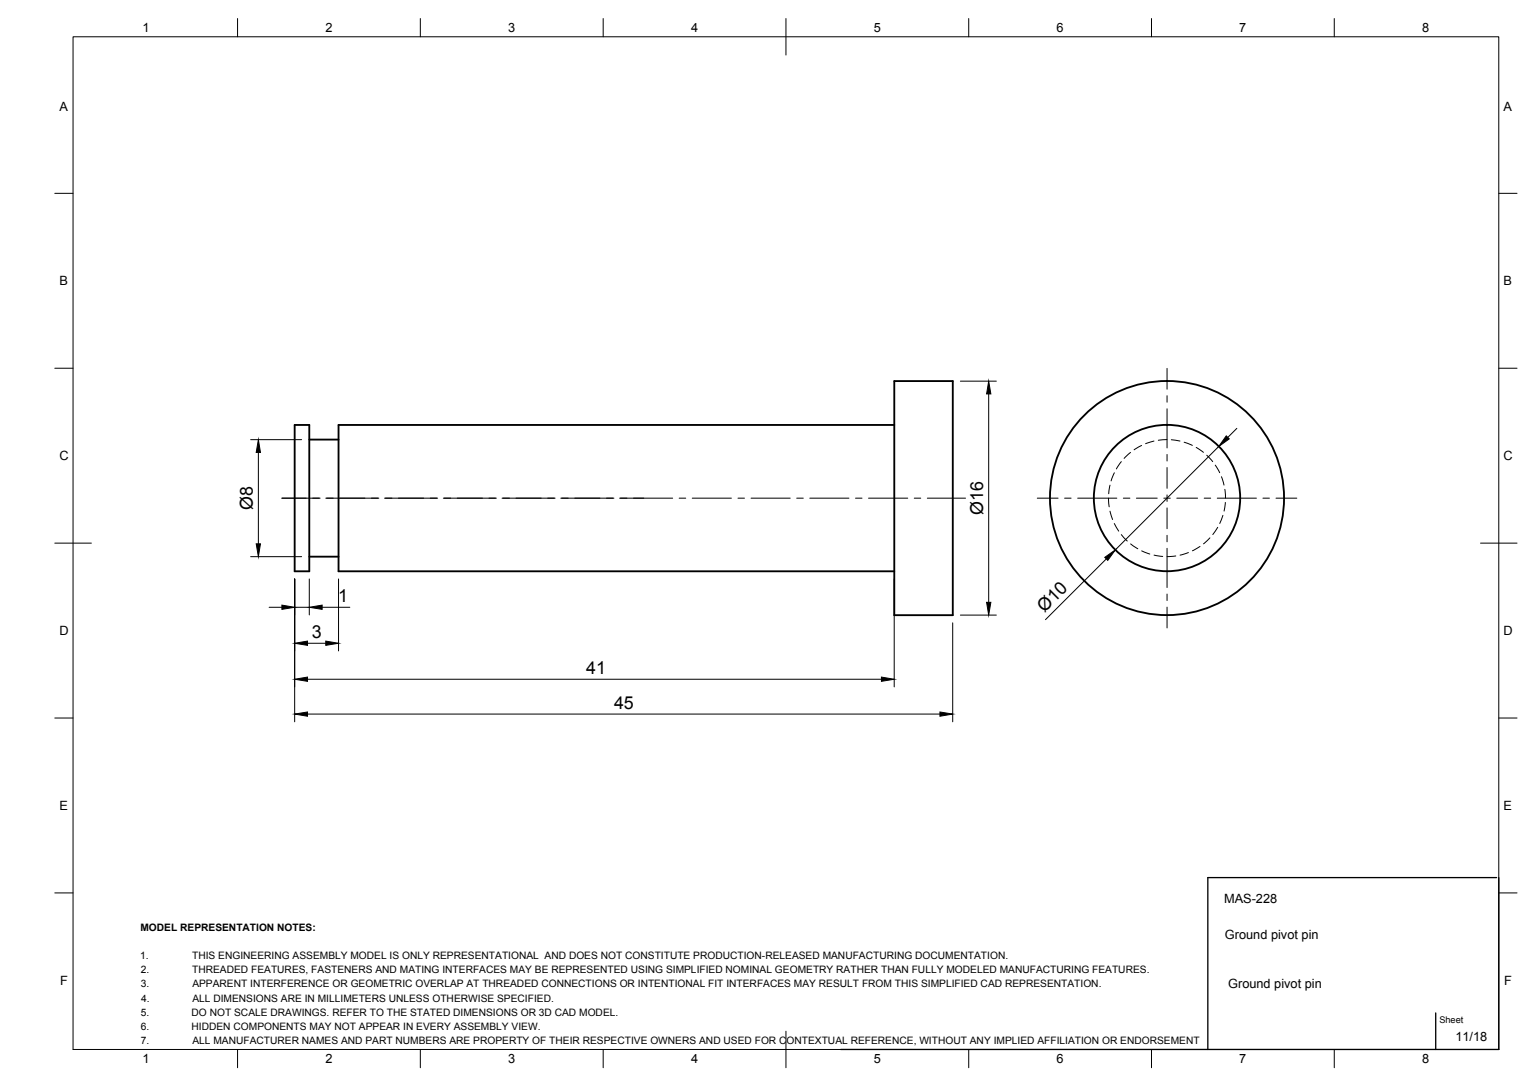
ISO-10303-21;
HEADER;
/* Generated by software containing ST-Developer
 * from STEP Tools, Inc. (www.steptools.com) 
 */

FILE_DESCRIPTION(
/* description */ ('Independent Peaucellier-Lipkin straight-line linkage. Radius arms 100
 mm, inversion-cell links 60 mm, crank radius and fixed-pivot spacing 
32 mm. Inversion constant 6400 mm squared, nominal output straight lin
e X=100 mm. Overhead bearing bridge clears the layered moving links. N
o accuracy or load rating assigned.'),
/* implementation_level */ '2;1');

FILE_NAME(
/* name */ 'Ground pivot pin.step',
/* time_stamp */ '2026-11-09T18:06:16-08:00',
/* author */ (''),
/* organization */ (''),
/* preprocessor_version */ 'ST-DEVELOPER v20.2',
/* originating_system */ 'Autodesk Translation Framework v15.17.0.0',
/* authorisation */ '');

FILE_SCHEMA (('AUTOMOTIVE_DESIGN { 1 0 10303 214 3 1 1 }'));
ENDSEC;

DATA;
#10=MECHANICAL_DESIGN_GEOMETRIC_PRESENTATION_REPRESENTATION('',(#289),#3581);
#255=SHAPE_REPRESENTATION_RELATIONSHIP('SRR','None',#3689,#272);
#272=ADVANCED_BREP_SHAPE_REPRESENTATION('',(#306),#3571);
#289=STYLED_ITEM('',(#3782),#306);
#306=MANIFOLD_SOLID_BREP('Body1',#1875);
#342=FACE_BOUND('',#613,.T.);
#343=FACE_BOUND('',#615,.T.);
#344=FACE_BOUND('',#618,.T.);
#392=PLANE('',#2176);
#393=PLANE('',#2178);
#394=PLANE('',#2182);
#395=PLANE('',#2187);
#396=PLANE('',#2189);
#474=FACE_OUTER_BOUND('',#611,.T.);
#475=FACE_OUTER_BOUND('',#612,.T.);
#476=FACE_OUTER_BOUND('',#614,.T.);
#477=FACE_OUTER_BOUND('',#616,.T.);
#478=FACE_OUTER_BOUND('',#617,.T.);
#479=FACE_OUTER_BOUND('',#619,.T.);
#480=FACE_OUTER_BOUND('',#620,.T.);
#481=FACE_OUTER_BOUND('',#621,.T.);
#482=FACE_OUTER_BOUND('',#622,.T.);
#611=EDGE_LOOP('',(#1526,#1527,#1528,#1529));
#612=EDGE_LOOP('',(#1530));
#613=EDGE_LOOP('',(#1531));
#614=EDGE_LOOP('',(#1532));
#615=EDGE_LOOP('',(#1533));
#616=EDGE_LOOP('',(#1534,#1535,#1536,#1537));
#617=EDGE_LOOP('',(#1538));
#618=EDGE_LOOP('',(#1539));
#619=EDGE_LOOP('',(#1540,#1541,#1542,#1543));
#620=EDGE_LOOP('',(#1544));
#621=EDGE_LOOP('',(#1545,#1546,#1547,#1548));
#622=EDGE_LOOP('',(#1549));
#758=LINE('',#3266,#856);
#759=LINE('',#3277,#857);
#760=LINE('',#3285,#858);
#761=LINE('',#3289,#859);
#856=VECTOR('',#2626,4.);
#857=VECTOR('',#2641,5.);
#858=VECTOR('',#2650,8.);
#859=VECTOR('',#2657,5.);
#933=CIRCLE('',#2174,4.);
#934=CIRCLE('',#2175,4.);
#935=CIRCLE('',#2177,5.);
#936=CIRCLE('',#2179,5.);
#937=CIRCLE('',#2181,5.);
#938=CIRCLE('',#2183,8.);
#939=CIRCLE('',#2184,5.);
#940=CIRCLE('',#2186,8.);
#1059=VERTEX_POINT('',#3263);
#1060=VERTEX_POINT('',#3265);
#1061=VERTEX_POINT('',#3269);
#1062=VERTEX_POINT('',#3272);
#1063=VERTEX_POINT('',#3275);
#1064=VERTEX_POINT('',#3279);
#1065=VERTEX_POINT('',#3281);
#1066=VERTEX_POINT('',#3284);
#1225=EDGE_CURVE('',#1059,#1059,#933,.T.);
#1226=EDGE_CURVE('',#1059,#1060,#758,.T.);
#1227=EDGE_CURVE('',#1060,#1060,#934,.T.);
#1228=EDGE_CURVE('',#1061,#1061,#935,.T.);
#1229=EDGE_CURVE('',#1062,#1062,#936,.T.);
#1230=EDGE_CURVE('',#1063,#1063,#937,.T.);
#1231=EDGE_CURVE('',#1063,#1062,#759,.T.);
#1232=EDGE_CURVE('',#1064,#1064,#938,.T.);
#1233=EDGE_CURVE('',#1065,#1065,#939,.T.);
#1234=EDGE_CURVE('',#1064,#1066,#760,.T.);
#1235=EDGE_CURVE('',#1066,#1066,#940,.T.);
#1236=EDGE_CURVE('',#1061,#1065,#761,.T.);
#1526=ORIENTED_EDGE('',*,*,#1225,.T.);
#1527=ORIENTED_EDGE('',*,*,#1226,.T.);
#1528=ORIENTED_EDGE('',*,*,#1227,.F.);
#1529=ORIENTED_EDGE('',*,*,#1226,.F.);
#1530=ORIENTED_EDGE('',*,*,#1228,.F.);
#1531=ORIENTED_EDGE('',*,*,#1225,.F.);
#1532=ORIENTED_EDGE('',*,*,#1229,.F.);
#1533=ORIENTED_EDGE('',*,*,#1227,.T.);
#1534=ORIENTED_EDGE('',*,*,#1230,.F.);
#1535=ORIENTED_EDGE('',*,*,#1231,.T.);
#1536=ORIENTED_EDGE('',*,*,#1229,.T.);
#1537=ORIENTED_EDGE('',*,*,#1231,.F.);
#1538=ORIENTED_EDGE('',*,*,#1232,.T.);
#1539=ORIENTED_EDGE('',*,*,#1233,.F.);
#1540=ORIENTED_EDGE('',*,*,#1232,.F.);
#1541=ORIENTED_EDGE('',*,*,#1234,.T.);
#1542=ORIENTED_EDGE('',*,*,#1235,.T.);
#1543=ORIENTED_EDGE('',*,*,#1234,.F.);
#1544=ORIENTED_EDGE('',*,*,#1235,.F.);
#1545=ORIENTED_EDGE('',*,*,#1228,.T.);
#1546=ORIENTED_EDGE('',*,*,#1236,.T.);
#1547=ORIENTED_EDGE('',*,*,#1233,.T.);
#1548=ORIENTED_EDGE('',*,*,#1236,.F.);
#1549=ORIENTED_EDGE('',*,*,#1230,.T.);
#1729=CYLINDRICAL_SURFACE('',#2173,4.);
#1730=CYLINDRICAL_SURFACE('',#2180,5.);
#1731=CYLINDRICAL_SURFACE('',#2185,8.);
#1732=CYLINDRICAL_SURFACE('',#2188,5.);
#1806=ADVANCED_FACE('',(#474),#1729,.T.);
#1807=ADVANCED_FACE('',(#475,#342),#392,.F.);
#1808=ADVANCED_FACE('',(#476,#343),#393,.F.);
#1809=ADVANCED_FACE('',(#477),#1730,.T.);
#1810=ADVANCED_FACE('',(#478,#344),#394,.T.);
#1811=ADVANCED_FACE('',(#479),#1731,.T.);
#1812=ADVANCED_FACE('',(#480),#395,.F.);
#1813=ADVANCED_FACE('',(#481),#1732,.T.);
#1814=ADVANCED_FACE('',(#482),#396,.T.);
#1875=CLOSED_SHELL('',(#1806,#1807,#1808,#1809,#1810,#1811,#1812,#1813,
#1814));
#2172=AXIS2_PLACEMENT_3D('',#3261,#2620,#2621);
#2173=AXIS2_PLACEMENT_3D('',#3262,#2622,#2623);
#2174=AXIS2_PLACEMENT_3D('',#3264,#2624,#2625);
#2175=AXIS2_PLACEMENT_3D('',#3267,#2627,#2628);
#2176=AXIS2_PLACEMENT_3D('',#3268,#2629,#2630);
#2177=AXIS2_PLACEMENT_3D('',#3270,#2631,#2632);
#2178=AXIS2_PLACEMENT_3D('',#3271,#2633,#2634);
#2179=AXIS2_PLACEMENT_3D('',#3273,#2635,#2636);
#2180=AXIS2_PLACEMENT_3D('',#3274,#2637,#2638);
#2181=AXIS2_PLACEMENT_3D('',#3276,#2639,#2640);
#2182=AXIS2_PLACEMENT_3D('',#3278,#2642,#2643);
#2183=AXIS2_PLACEMENT_3D('',#3280,#2644,#2645);
#2184=AXIS2_PLACEMENT_3D('',#3282,#2646,#2647);
#2185=AXIS2_PLACEMENT_3D('',#3283,#2648,#2649);
#2186=AXIS2_PLACEMENT_3D('',#3286,#2651,#2652);
#2187=AXIS2_PLACEMENT_3D('',#3287,#2653,#2654);
#2188=AXIS2_PLACEMENT_3D('',#3288,#2655,#2656);
#2189=AXIS2_PLACEMENT_3D('',#3290,#2658,#2659);
#2620=DIRECTION('axis',(0.,0.,1.));
#2621=DIRECTION('refdir',(1.,0.,0.));
#2622=DIRECTION('center_axis',(0.,0.,1.));
#2623=DIRECTION('ref_axis',(1.,0.,0.));
#2624=DIRECTION('center_axis',(0.,0.,1.));
#2625=DIRECTION('ref_axis',(1.,0.,0.));
#2626=DIRECTION('',(0.,0.,1.));
#2627=DIRECTION('center_axis',(0.,0.,1.));
#2628=DIRECTION('ref_axis',(1.,0.,0.));
#2629=DIRECTION('center_axis',(0.,0.,-1.));
#2630=DIRECTION('ref_axis',(-1.,0.,0.));
#2631=DIRECTION('center_axis',(0.,0.,-1.));
#2632=DIRECTION('ref_axis',(1.,0.,0.));
#2633=DIRECTION('center_axis',(0.,0.,1.));
#2634=DIRECTION('ref_axis',(1.,0.,0.));
#2635=DIRECTION('center_axis',(0.,0.,1.));
#2636=DIRECTION('ref_axis',(1.,0.,0.));
#2637=DIRECTION('center_axis',(0.,0.,1.));
#2638=DIRECTION('ref_axis',(1.,0.,0.));
#2639=DIRECTION('center_axis',(0.,0.,1.));
#2640=DIRECTION('ref_axis',(1.,0.,0.));
#2641=DIRECTION('',(0.,0.,-1.));
#2642=DIRECTION('center_axis',(0.,0.,1.));
#2643=DIRECTION('ref_axis',(1.,0.,0.));
#2644=DIRECTION('center_axis',(0.,0.,1.));
#2645=DIRECTION('ref_axis',(1.,0.,0.));
#2646=DIRECTION('center_axis',(0.,0.,1.));
#2647=DIRECTION('ref_axis',(1.,0.,0.));
#2648=DIRECTION('center_axis',(0.,0.,1.));
#2649=DIRECTION('ref_axis',(1.,0.,0.));
#2650=DIRECTION('',(0.,0.,-1.));
#2651=DIRECTION('center_axis',(0.,0.,1.));
#2652=DIRECTION('ref_axis',(1.,0.,0.));
#2653=DIRECTION('center_axis',(0.,0.,1.));
#2654=DIRECTION('ref_axis',(1.,0.,0.));
#2655=DIRECTION('center_axis',(0.,0.,1.));
#2656=DIRECTION('ref_axis',(1.,0.,0.));
#2657=DIRECTION('',(0.,0.,-1.));
#2658=DIRECTION('center_axis',(0.,0.,1.));
#2659=DIRECTION('ref_axis',(1.,0.,0.));
#3261=CARTESIAN_POINT('',(0.,0.,0.));
#3262=CARTESIAN_POINT('Origin',(0.,0.,39.));
#3263=CARTESIAN_POINT('',(-4.,-4.89858719658941E-16,38.));
#3264=CARTESIAN_POINT('Origin',(0.,0.,38.));
#3265=CARTESIAN_POINT('',(-4.,-4.89858719658941E-16,40.));
#3266=CARTESIAN_POINT('',(-4.,-4.89858719658941E-16,39.));
#3267=CARTESIAN_POINT('Origin',(0.,0.,40.));
#3268=CARTESIAN_POINT('Origin',(8.,0.,38.));
#3269=CARTESIAN_POINT('',(-5.,6.12323399573677E-16,38.));
#3270=CARTESIAN_POINT('Origin',(0.,0.,38.));
#3271=CARTESIAN_POINT('Origin',(4.,0.,40.));
#3272=CARTESIAN_POINT('',(-5.,-6.12323399573677E-16,40.));
#3273=CARTESIAN_POINT('Origin',(0.,0.,40.));
#3274=CARTESIAN_POINT('Origin',(0.,0.,0.));
#3275=CARTESIAN_POINT('',(-5.,-6.12323399573677E-16,41.));
#3276=CARTESIAN_POINT('Origin',(0.,0.,41.));
#3277=CARTESIAN_POINT('',(-5.,-6.12323399573677E-16,0.));
#3278=CARTESIAN_POINT('Origin',(0.,0.,0.));
#3279=CARTESIAN_POINT('',(-8.,-9.79717439317883E-16,0.));
#3280=CARTESIAN_POINT('Origin',(0.,0.,0.));
#3281=CARTESIAN_POINT('',(-5.,-6.12323399573677E-16,0.));
#3282=CARTESIAN_POINT('Origin',(0.,0.,0.));
#3283=CARTESIAN_POINT('Origin',(0.,0.,-4.));
#3284=CARTESIAN_POINT('',(-8.,-9.79717439317883E-16,-4.));
#3285=CARTESIAN_POINT('',(-8.,-9.79717439317883E-16,-4.));
#3286=CARTESIAN_POINT('Origin',(0.,0.,-4.));
#3287=CARTESIAN_POINT('Origin',(0.,0.,-4.));
#3288=CARTESIAN_POINT('Origin',(0.,0.,0.));
#3289=CARTESIAN_POINT('',(-5.,-6.12323399573677E-16,0.));
#3290=CARTESIAN_POINT('Origin',(0.,0.,41.));
#3552=UNCERTAINTY_MEASURE_WITH_UNIT(LENGTH_MEASURE(0.01),#3582,
'DISTANCE_ACCURACY_VALUE',
'Maximum model space distance between geometric entities at asserted c
onnectivities');
#3562=UNCERTAINTY_MEASURE_WITH_UNIT(LENGTH_MEASURE(0.01),#3582,
'DISTANCE_ACCURACY_VALUE',
'Maximum model space distance between geometric entities at asserted c
onnectivities');
#3571=(
GEOMETRIC_REPRESENTATION_CONTEXT(3)
GLOBAL_UNCERTAINTY_ASSIGNED_CONTEXT((#3552))
GLOBAL_UNIT_ASSIGNED_CONTEXT((#3582,#3584,#3585))
REPRESENTATION_CONTEXT('','3D')
);
#3581=(
GEOMETRIC_REPRESENTATION_CONTEXT(3)
GLOBAL_UNCERTAINTY_ASSIGNED_CONTEXT((#3562))
GLOBAL_UNIT_ASSIGNED_CONTEXT((#3582,#3584,#3585))
REPRESENTATION_CONTEXT('','3D')
);
#3582=(
LENGTH_UNIT()
NAMED_UNIT(*)
SI_UNIT(.MILLI.,.METRE.)
);
#3584=(
NAMED_UNIT(*)
PLANE_ANGLE_UNIT()
SI_UNIT($,.RADIAN.)
);
#3585=(
NAMED_UNIT(*)
SI_UNIT($,.STERADIAN.)
SOLID_ANGLE_UNIT()
);
#3594=SHAPE_DEFINITION_REPRESENTATION(#3612,#3689);
#3612=PRODUCT_DEFINITION_SHAPE('',$,#3708);
#3689=SHAPE_REPRESENTATION('',(#2172),#3571);
#3699=PRODUCT_DEFINITION_CONTEXT('part definition',#3755,'design');
#3708=PRODUCT_DEFINITION('Ground pivot pin','Ground pivot pin',#3726,#3699);
#3726=PRODUCT_DEFINITION_FORMATION('',$,#3765);
#3755=APPLICATION_CONTEXT(
'Core Data for Automotive Mechanical Design Process');
#3756=PRODUCT_CONTEXT('part definition',#3755,'mechanical');
#3765=PRODUCT('Ground pivot pin','Ground pivot pin',$,(#3756));
#3782=PRESENTATION_STYLE_ASSIGNMENT((#3795));
#3795=SURFACE_STYLE_USAGE(.BOTH.,#3808);
#3808=SURFACE_SIDE_STYLE('',(#3821));
#3821=SURFACE_STYLE_FILL_AREA(#3834);
#3834=FILL_AREA_STYLE('Pivot gray',(#3847));
#3847=FILL_AREA_STYLE_COLOUR('Pivot gray',#3860);
#3860=COLOUR_RGB('Pivot gray',0.407843137254902,0.447058823529412,0.498039215686275);
ENDSEC;
END-ISO-10303-21;
